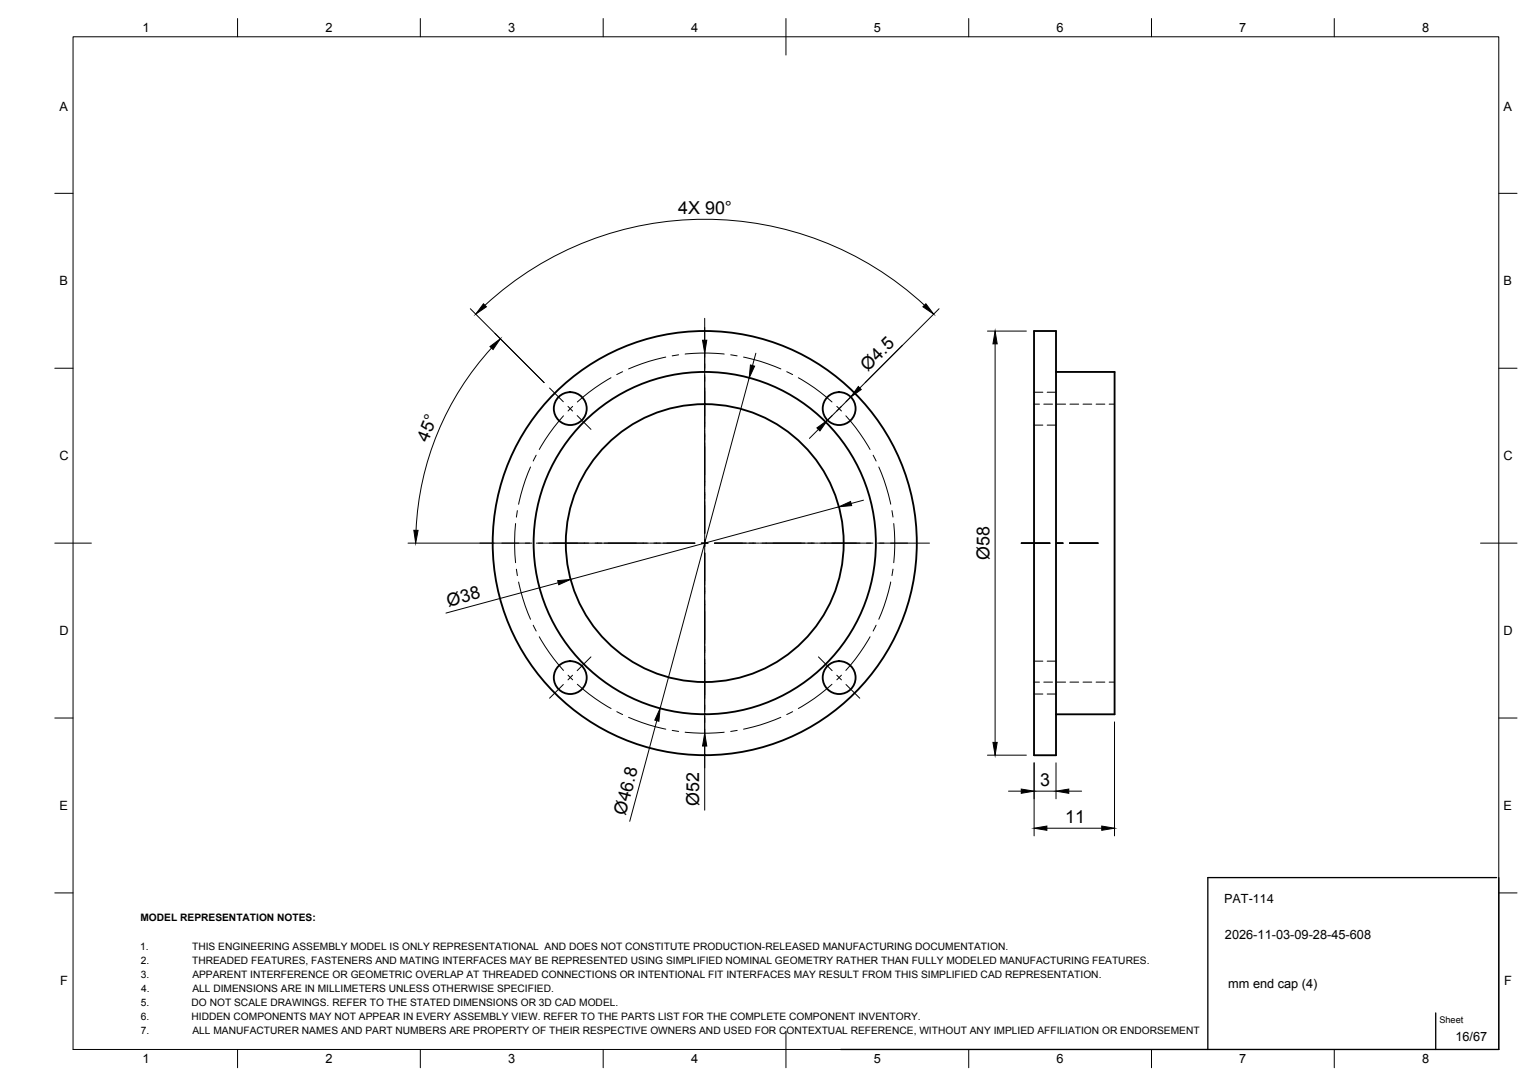
ISO-10303-21;
HEADER;
/* Generated by software containing ST-Developer
 * from STEP Tools, Inc. (www.steptools.com) 
 */

FILE_DESCRIPTION(
/* description */ ('Two-stage gear reducer in split housing'),
/* implementation_level */ '2;1');

FILE_NAME(
/* name */ 'mm end cap (4).step',
/* time_stamp */ '2026-10-28T03:22:31-07:00',
/* author */ (''),
/* organization */ (''),
/* preprocessor_version */ 'ST-DEVELOPER v20.2',
/* originating_system */ 'Autodesk Translation Framework v15.17.0.0',
/* authorisation */ '');

FILE_SCHEMA (('AUTOMOTIVE_DESIGN { 1 0 10303 214 3 1 1 }'));
ENDSEC;

DATA;
#10=MECHANICAL_DESIGN_GEOMETRIC_PRESENTATION_REPRESENTATION('',(#1245),#73366);
#1133=SHAPE_REPRESENTATION_RELATIONSHIP('SRR','None',#73620,#1189);
#1189=ADVANCED_BREP_SHAPE_REPRESENTATION('',(#1316),#73316);
#1245=STYLED_ITEM('',(#74002),#1316);
#1316=MANIFOLD_SOLID_BREP('Body1',#16133);
#1488=FACE_BOUND('',#3275,.T.);
#1489=FACE_BOUND('',#3279,.T.);
#1490=FACE_BOUND('',#3280,.T.);
#1491=FACE_BOUND('',#3281,.T.);
#1492=FACE_BOUND('',#3282,.T.);
#1493=FACE_BOUND('',#3283,.T.);
#1494=FACE_BOUND('',#3285,.T.);
#1495=FACE_BOUND('',#3286,.T.);
#1496=FACE_BOUND('',#3287,.T.);
#1497=FACE_BOUND('',#3288,.T.);
#1498=FACE_BOUND('',#3289,.T.);
#1720=PLANE('',#17325);
#1721=PLANE('',#17332);
#1722=PLANE('',#17333);
#2242=FACE_OUTER_BOUND('',#3269,.T.);
#2243=FACE_OUTER_BOUND('',#3270,.T.);
#2244=FACE_OUTER_BOUND('',#3271,.T.);
#2245=FACE_OUTER_BOUND('',#3272,.T.);
#2246=FACE_OUTER_BOUND('',#3273,.T.);
#2247=FACE_OUTER_BOUND('',#3274,.T.);
#2248=FACE_OUTER_BOUND('',#3276,.T.);
#2249=FACE_OUTER_BOUND('',#3277,.T.);
#2250=FACE_OUTER_BOUND('',#3278,.T.);
#2251=FACE_OUTER_BOUND('',#3284,.T.);
#3269=EDGE_LOOP('',(#11575,#11576,#11577,#11578));
#3270=EDGE_LOOP('',(#11579,#11580,#11581,#11582));
#3271=EDGE_LOOP('',(#11583,#11584,#11585,#11586));
#3272=EDGE_LOOP('',(#11587,#11588,#11589,#11590));
#3273=EDGE_LOOP('',(#11591,#11592,#11593,#11594));
#3274=EDGE_LOOP('',(#11595));
#3275=EDGE_LOOP('',(#11596));
#3276=EDGE_LOOP('',(#11597,#11598,#11599,#11600));
#3277=EDGE_LOOP('',(#11601,#11602,#11603,#11604));
#3278=EDGE_LOOP('',(#11605));
#3279=EDGE_LOOP('',(#11606));
#3280=EDGE_LOOP('',(#11607));
#3281=EDGE_LOOP('',(#11608));
#3282=EDGE_LOOP('',(#11609));
#3283=EDGE_LOOP('',(#11610));
#3284=EDGE_LOOP('',(#11611));
#3285=EDGE_LOOP('',(#11612));
#3286=EDGE_LOOP('',(#11613));
#3287=EDGE_LOOP('',(#11614));
#3288=EDGE_LOOP('',(#11615));
#3289=EDGE_LOOP('',(#11616));
#4346=LINE('',#23922,#5370);
#4347=LINE('',#23928,#5371);
#4348=LINE('',#23934,#5372);
#4349=LINE('',#23940,#5373);
#4350=LINE('',#23946,#5374);
#4351=LINE('',#23953,#5375);
#4352=LINE('',#23959,#5376);
#5370=VECTOR('',#19748,0.225);
#5371=VECTOR('',#19755,0.225);
#5372=VECTOR('',#19762,0.225);
#5373=VECTOR('',#19769,0.225);
#5374=VECTOR('',#19776,2.34);
#5375=VECTOR('',#19785,1.9);
#5376=VECTOR('',#19792,2.9);
#6348=CIRCLE('',#17311,0.225);
#6349=CIRCLE('',#17312,0.225);
#6350=CIRCLE('',#17314,0.225);
#6351=CIRCLE('',#17315,0.225);
#6352=CIRCLE('',#17317,0.225);
#6353=CIRCLE('',#17318,0.225);
#6354=CIRCLE('',#17320,0.225);
#6355=CIRCLE('',#17321,0.225);
#6356=CIRCLE('',#17323,2.34);
#6357=CIRCLE('',#17324,2.34);
#6358=CIRCLE('',#17326,1.9);
#6359=CIRCLE('',#17328,1.9);
#6360=CIRCLE('',#17330,2.9);
#6361=CIRCLE('',#17331,2.9);
#7180=VERTEX_POINT('',#23919);
#7181=VERTEX_POINT('',#23921);
#7182=VERTEX_POINT('',#23925);
#7183=VERTEX_POINT('',#23927);
#7184=VERTEX_POINT('',#23931);
#7185=VERTEX_POINT('',#23933);
#7186=VERTEX_POINT('',#23937);
#7187=VERTEX_POINT('',#23939);
#7188=VERTEX_POINT('',#23943);
#7189=VERTEX_POINT('',#23945);
#7190=VERTEX_POINT('',#23949);
#7191=VERTEX_POINT('',#23952);
#7192=VERTEX_POINT('',#23956);
#7193=VERTEX_POINT('',#23958);
#8841=EDGE_CURVE('',#7180,#7180,#6348,.T.);
#8842=EDGE_CURVE('',#7180,#7181,#4346,.T.);
#8843=EDGE_CURVE('',#7181,#7181,#6349,.T.);
#8844=EDGE_CURVE('',#7182,#7182,#6350,.T.);
#8845=EDGE_CURVE('',#7182,#7183,#4347,.T.);
#8846=EDGE_CURVE('',#7183,#7183,#6351,.T.);
#8847=EDGE_CURVE('',#7184,#7184,#6352,.T.);
#8848=EDGE_CURVE('',#7184,#7185,#4348,.T.);
#8849=EDGE_CURVE('',#7185,#7185,#6353,.T.);
#8850=EDGE_CURVE('',#7186,#7186,#6354,.T.);
#8851=EDGE_CURVE('',#7186,#7187,#4349,.T.);
#8852=EDGE_CURVE('',#7187,#7187,#6355,.T.);
#8853=EDGE_CURVE('',#7188,#7188,#6356,.T.);
#8854=EDGE_CURVE('',#7188,#7189,#4350,.T.);
#8855=EDGE_CURVE('',#7189,#7189,#6357,.T.);
#8856=EDGE_CURVE('',#7190,#7190,#6358,.T.);
#8857=EDGE_CURVE('',#7190,#7191,#4351,.T.);
#8858=EDGE_CURVE('',#7191,#7191,#6359,.T.);
#8859=EDGE_CURVE('',#7192,#7192,#6360,.T.);
#8860=EDGE_CURVE('',#7192,#7193,#4352,.T.);
#8861=EDGE_CURVE('',#7193,#7193,#6361,.T.);
#11575=ORIENTED_EDGE('',*,*,#8841,.F.);
#11576=ORIENTED_EDGE('',*,*,#8842,.T.);
#11577=ORIENTED_EDGE('',*,*,#8843,.F.);
#11578=ORIENTED_EDGE('',*,*,#8842,.F.);
#11579=ORIENTED_EDGE('',*,*,#8844,.F.);
#11580=ORIENTED_EDGE('',*,*,#8845,.T.);
#11581=ORIENTED_EDGE('',*,*,#8846,.F.);
#11582=ORIENTED_EDGE('',*,*,#8845,.F.);
#11583=ORIENTED_EDGE('',*,*,#8847,.F.);
#11584=ORIENTED_EDGE('',*,*,#8848,.T.);
#11585=ORIENTED_EDGE('',*,*,#8849,.F.);
#11586=ORIENTED_EDGE('',*,*,#8848,.F.);
#11587=ORIENTED_EDGE('',*,*,#8850,.F.);
#11588=ORIENTED_EDGE('',*,*,#8851,.T.);
#11589=ORIENTED_EDGE('',*,*,#8852,.F.);
#11590=ORIENTED_EDGE('',*,*,#8851,.F.);
#11591=ORIENTED_EDGE('',*,*,#8853,.F.);
#11592=ORIENTED_EDGE('',*,*,#8854,.T.);
#11593=ORIENTED_EDGE('',*,*,#8855,.F.);
#11594=ORIENTED_EDGE('',*,*,#8854,.F.);
#11595=ORIENTED_EDGE('',*,*,#8853,.T.);
#11596=ORIENTED_EDGE('',*,*,#8856,.T.);
#11597=ORIENTED_EDGE('',*,*,#8856,.F.);
#11598=ORIENTED_EDGE('',*,*,#8857,.T.);
#11599=ORIENTED_EDGE('',*,*,#8858,.T.);
#11600=ORIENTED_EDGE('',*,*,#8857,.F.);
#11601=ORIENTED_EDGE('',*,*,#8859,.F.);
#11602=ORIENTED_EDGE('',*,*,#8860,.T.);
#11603=ORIENTED_EDGE('',*,*,#8861,.T.);
#11604=ORIENTED_EDGE('',*,*,#8860,.F.);
#11605=ORIENTED_EDGE('',*,*,#8859,.T.);
#11606=ORIENTED_EDGE('',*,*,#8855,.T.);
#11607=ORIENTED_EDGE('',*,*,#8852,.T.);
#11608=ORIENTED_EDGE('',*,*,#8849,.T.);
#11609=ORIENTED_EDGE('',*,*,#8846,.T.);
#11610=ORIENTED_EDGE('',*,*,#8843,.T.);
#11611=ORIENTED_EDGE('',*,*,#8861,.F.);
#11612=ORIENTED_EDGE('',*,*,#8858,.F.);
#11613=ORIENTED_EDGE('',*,*,#8850,.T.);
#11614=ORIENTED_EDGE('',*,*,#8847,.T.);
#11615=ORIENTED_EDGE('',*,*,#8844,.T.);
#11616=ORIENTED_EDGE('',*,*,#8841,.T.);
#15029=CYLINDRICAL_SURFACE('',#17310,0.225);
#15030=CYLINDRICAL_SURFACE('',#17313,0.225);
#15031=CYLINDRICAL_SURFACE('',#17316,0.225);
#15032=CYLINDRICAL_SURFACE('',#17319,0.225);
#15033=CYLINDRICAL_SURFACE('',#17322,2.34);
#15034=CYLINDRICAL_SURFACE('',#17327,1.9);
#15035=CYLINDRICAL_SURFACE('',#17329,2.9);
#15449=ADVANCED_FACE('',(#2242),#15029,.F.);
#15450=ADVANCED_FACE('',(#2243),#15030,.F.);
#15451=ADVANCED_FACE('',(#2244),#15031,.F.);
#15452=ADVANCED_FACE('',(#2245),#15032,.F.);
#15453=ADVANCED_FACE('',(#2246),#15033,.T.);
#15454=ADVANCED_FACE('',(#2247,#1488),#1720,.T.);
#15455=ADVANCED_FACE('',(#2248),#15034,.F.);
#15456=ADVANCED_FACE('',(#2249),#15035,.T.);
#15457=ADVANCED_FACE('',(#2250,#1489,#1490,#1491,#1492,#1493),#1721,.T.);
#15458=ADVANCED_FACE('',(#2251,#1494,#1495,#1496,#1497,#1498),#1722,.F.);
#16133=CLOSED_SHELL('',(#15449,#15450,#15451,#15452,#15453,#15454,#15455,
#15456,#15457,#15458));
#17309=AXIS2_PLACEMENT_3D('',#23917,#19742,#19743);
#17310=AXIS2_PLACEMENT_3D('',#23918,#19744,#19745);
#17311=AXIS2_PLACEMENT_3D('',#23920,#19746,#19747);
#17312=AXIS2_PLACEMENT_3D('',#23923,#19749,#19750);
#17313=AXIS2_PLACEMENT_3D('',#23924,#19751,#19752);
#17314=AXIS2_PLACEMENT_3D('',#23926,#19753,#19754);
#17315=AXIS2_PLACEMENT_3D('',#23929,#19756,#19757);
#17316=AXIS2_PLACEMENT_3D('',#23930,#19758,#19759);
#17317=AXIS2_PLACEMENT_3D('',#23932,#19760,#19761);
#17318=AXIS2_PLACEMENT_3D('',#23935,#19763,#19764);
#17319=AXIS2_PLACEMENT_3D('',#23936,#19765,#19766);
#17320=AXIS2_PLACEMENT_3D('',#23938,#19767,#19768);
#17321=AXIS2_PLACEMENT_3D('',#23941,#19770,#19771);
#17322=AXIS2_PLACEMENT_3D('',#23942,#19772,#19773);
#17323=AXIS2_PLACEMENT_3D('',#23944,#19774,#19775);
#17324=AXIS2_PLACEMENT_3D('',#23947,#19777,#19778);
#17325=AXIS2_PLACEMENT_3D('',#23948,#19779,#19780);
#17326=AXIS2_PLACEMENT_3D('',#23950,#19781,#19782);
#17327=AXIS2_PLACEMENT_3D('',#23951,#19783,#19784);
#17328=AXIS2_PLACEMENT_3D('',#23954,#19786,#19787);
#17329=AXIS2_PLACEMENT_3D('',#23955,#19788,#19789);
#17330=AXIS2_PLACEMENT_3D('',#23957,#19790,#19791);
#17331=AXIS2_PLACEMENT_3D('',#23960,#19793,#19794);
#17332=AXIS2_PLACEMENT_3D('',#23961,#19795,#19796);
#17333=AXIS2_PLACEMENT_3D('',#23962,#19797,#19798);
#19742=DIRECTION('axis',(0.,0.,1.));
#19743=DIRECTION('refdir',(1.,0.,0.));
#19744=DIRECTION('center_axis',(0.,1.,0.));
#19745=DIRECTION('ref_axis',(1.,0.,0.));
#19746=DIRECTION('center_axis',(0.,1.,0.));
#19747=DIRECTION('ref_axis',(1.,0.,0.));
#19748=DIRECTION('',(0.,1.,0.));
#19749=DIRECTION('center_axis',(0.,-1.,0.));
#19750=DIRECTION('ref_axis',(1.,0.,0.));
#19751=DIRECTION('center_axis',(0.,1.,0.));
#19752=DIRECTION('ref_axis',(1.,0.,0.));
#19753=DIRECTION('center_axis',(0.,1.,0.));
#19754=DIRECTION('ref_axis',(1.,0.,0.));
#19755=DIRECTION('',(0.,1.,0.));
#19756=DIRECTION('center_axis',(0.,-1.,0.));
#19757=DIRECTION('ref_axis',(1.,0.,0.));
#19758=DIRECTION('center_axis',(0.,1.,0.));
#19759=DIRECTION('ref_axis',(1.,0.,0.));
#19760=DIRECTION('center_axis',(0.,1.,0.));
#19761=DIRECTION('ref_axis',(1.,0.,0.));
#19762=DIRECTION('',(0.,1.,0.));
#19763=DIRECTION('center_axis',(0.,-1.,0.));
#19764=DIRECTION('ref_axis',(1.,0.,0.));
#19765=DIRECTION('center_axis',(0.,1.,0.));
#19766=DIRECTION('ref_axis',(1.,0.,0.));
#19767=DIRECTION('center_axis',(0.,1.,0.));
#19768=DIRECTION('ref_axis',(1.,0.,0.));
#19769=DIRECTION('',(0.,1.,0.));
#19770=DIRECTION('center_axis',(0.,-1.,0.));
#19771=DIRECTION('ref_axis',(1.,0.,0.));
#19772=DIRECTION('center_axis',(0.,1.,0.));
#19773=DIRECTION('ref_axis',(1.,0.,0.));
#19774=DIRECTION('center_axis',(0.,1.,0.));
#19775=DIRECTION('ref_axis',(1.,0.,0.));
#19776=DIRECTION('',(0.,-1.,0.));
#19777=DIRECTION('center_axis',(0.,-1.,0.));
#19778=DIRECTION('ref_axis',(1.,0.,0.));
#19779=DIRECTION('center_axis',(0.,1.,0.));
#19780=DIRECTION('ref_axis',(1.,0.,0.));
#19781=DIRECTION('center_axis',(0.,-1.,0.));
#19782=DIRECTION('ref_axis',(1.,0.,0.));
#19783=DIRECTION('center_axis',(0.,1.,0.));
#19784=DIRECTION('ref_axis',(1.,0.,0.));
#19785=DIRECTION('',(0.,-1.,0.));
#19786=DIRECTION('center_axis',(0.,-1.,0.));
#19787=DIRECTION('ref_axis',(1.,0.,0.));
#19788=DIRECTION('center_axis',(0.,1.,0.));
#19789=DIRECTION('ref_axis',(1.,0.,0.));
#19790=DIRECTION('center_axis',(0.,1.,0.));
#19791=DIRECTION('ref_axis',(1.,0.,0.));
#19792=DIRECTION('',(0.,-1.,0.));
#19793=DIRECTION('center_axis',(0.,1.,0.));
#19794=DIRECTION('ref_axis',(1.,0.,0.));
#19795=DIRECTION('center_axis',(0.,1.,0.));
#19796=DIRECTION('ref_axis',(1.,0.,0.));
#19797=DIRECTION('center_axis',(0.,1.,0.));
#19798=DIRECTION('ref_axis',(1.,0.,0.));
#23917=CARTESIAN_POINT('',(0.,0.,0.));
#23918=CARTESIAN_POINT('Origin',(10.161522368915,-7.9,8.16152236891498));
#23919=CARTESIAN_POINT('',(9.93652236891498,-7.8,8.16152236891498));
#23920=CARTESIAN_POINT('Origin',(10.161522368915,-7.8,8.16152236891498));
#23921=CARTESIAN_POINT('',(9.93652236891498,-7.5,8.16152236891498));
#23922=CARTESIAN_POINT('',(9.93652236891498,-7.9,8.16152236891498));
#23923=CARTESIAN_POINT('Origin',(10.161522368915,-7.5,8.16152236891498));
#23924=CARTESIAN_POINT('Origin',(10.161522368915,-7.9,11.838477631085));
#23925=CARTESIAN_POINT('',(9.93652236891498,-7.8,11.838477631085));
#23926=CARTESIAN_POINT('Origin',(10.161522368915,-7.8,11.838477631085));
#23927=CARTESIAN_POINT('',(9.93652236891498,-7.5,11.838477631085));
#23928=CARTESIAN_POINT('',(9.93652236891498,-7.9,11.838477631085));
#23929=CARTESIAN_POINT('Origin',(10.161522368915,-7.5,11.838477631085));
#23930=CARTESIAN_POINT('Origin',(13.838477631085,-7.9,11.838477631085));
#23931=CARTESIAN_POINT('',(13.613477631085,-7.8,11.838477631085));
#23932=CARTESIAN_POINT('Origin',(13.838477631085,-7.8,11.838477631085));
#23933=CARTESIAN_POINT('',(13.613477631085,-7.5,11.838477631085));
#23934=CARTESIAN_POINT('',(13.613477631085,-7.9,11.838477631085));
#23935=CARTESIAN_POINT('Origin',(13.838477631085,-7.5,11.838477631085));
#23936=CARTESIAN_POINT('Origin',(13.838477631085,-7.9,8.16152236891498));
#23937=CARTESIAN_POINT('',(13.613477631085,-7.8,8.16152236891498));
#23938=CARTESIAN_POINT('Origin',(13.838477631085,-7.8,8.16152236891498));
#23939=CARTESIAN_POINT('',(13.613477631085,-7.5,8.16152236891498));
#23940=CARTESIAN_POINT('',(13.613477631085,-7.9,8.16152236891498));
#23941=CARTESIAN_POINT('Origin',(13.838477631085,-7.5,8.16152236891498));
#23942=CARTESIAN_POINT('Origin',(12.,-7.5,10.));
#23943=CARTESIAN_POINT('',(9.66,-6.7,10.));
#23944=CARTESIAN_POINT('Origin',(12.,-6.7,10.));
#23945=CARTESIAN_POINT('',(9.66,-7.5,10.));
#23946=CARTESIAN_POINT('',(9.66,-7.5,10.));
#23947=CARTESIAN_POINT('Origin',(12.,-7.5,10.));
#23948=CARTESIAN_POINT('Origin',(12.,-6.7,10.));
#23949=CARTESIAN_POINT('',(10.1,-6.7,10.));
#23950=CARTESIAN_POINT('Origin',(12.,-6.7,10.));
#23951=CARTESIAN_POINT('Origin',(12.,-7.8,10.));
#23952=CARTESIAN_POINT('',(10.1,-7.8,10.));
#23953=CARTESIAN_POINT('',(10.1,-7.8,10.));
#23954=CARTESIAN_POINT('Origin',(12.,-7.8,10.));
#23955=CARTESIAN_POINT('Origin',(12.,-7.8,10.));
#23956=CARTESIAN_POINT('',(9.1,-7.5,10.));
#23957=CARTESIAN_POINT('Origin',(12.,-7.5,10.));
#23958=CARTESIAN_POINT('',(9.1,-7.8,10.));
#23959=CARTESIAN_POINT('',(9.1,-7.8,10.));
#23960=CARTESIAN_POINT('Origin',(12.,-7.8,10.));
#23961=CARTESIAN_POINT('Origin',(12.,-7.5,10.));
#23962=CARTESIAN_POINT('Origin',(12.,-7.8,10.));
#73252=UNCERTAINTY_MEASURE_WITH_UNIT(LENGTH_MEASURE(0.001),#73367,
'DISTANCE_ACCURACY_VALUE',
'Maximum model space distance between geometric entities at asserted c
onnectivities');
#73302=UNCERTAINTY_MEASURE_WITH_UNIT(LENGTH_MEASURE(0.001),#73367,
'DISTANCE_ACCURACY_VALUE',
'Maximum model space distance between geometric entities at asserted c
onnectivities');
#73316=(
GEOMETRIC_REPRESENTATION_CONTEXT(3)
GLOBAL_UNCERTAINTY_ASSIGNED_CONTEXT((#73252))
GLOBAL_UNIT_ASSIGNED_CONTEXT((#73367,#73369,#73370))
REPRESENTATION_CONTEXT('','3D')
);
#73366=(
GEOMETRIC_REPRESENTATION_CONTEXT(3)
GLOBAL_UNCERTAINTY_ASSIGNED_CONTEXT((#73302))
GLOBAL_UNIT_ASSIGNED_CONTEXT((#73367,#73369,#73370))
REPRESENTATION_CONTEXT('','3D')
);
#73367=(
LENGTH_UNIT()
NAMED_UNIT(*)
SI_UNIT(.CENTI.,.METRE.)
);
#73369=(
NAMED_UNIT(*)
PLANE_ANGLE_UNIT()
SI_UNIT($,.RADIAN.)
);
#73370=(
NAMED_UNIT(*)
SI_UNIT($,.STERADIAN.)
SOLID_ANGLE_UNIT()
);
#73384=SHAPE_DEFINITION_REPRESENTATION(#73447,#73620);
#73447=PRODUCT_DEFINITION_SHAPE('',$,#73684);
#73620=SHAPE_REPRESENTATION('',(#17309),#73316);
#73670=PRODUCT_DEFINITION_CONTEXT('part definition',#73861,'design');
#73684=PRODUCT_DEFINITION('mm end cap (4)','mm end cap (4)',#73747,#73670);
#73747=PRODUCT_DEFINITION_FORMATION('',$,#73876);
#73861=APPLICATION_CONTEXT(
'Core Data for Automotive Mechanical Design Process');
#73862=PRODUCT_CONTEXT('part definition',#73861,'mechanical');
#73876=PRODUCT('mm end cap (4)','mm end cap (4)','mm end cap (4)',(#73862));
#73996=COLOUR_RGB('Off White',0.89,0.88,0.83);
#73997=FILL_AREA_STYLE_COLOUR('',#73996);
#73998=FILL_AREA_STYLE('',(#73997));
#73999=SURFACE_STYLE_FILL_AREA(#73998);
#74000=SURFACE_SIDE_STYLE('',(#73999));
#74001=SURFACE_STYLE_USAGE(.BOTH.,#74000);
#74002=PRESENTATION_STYLE_ASSIGNMENT((#74001));
ENDSEC;
END-ISO-10303-21;
